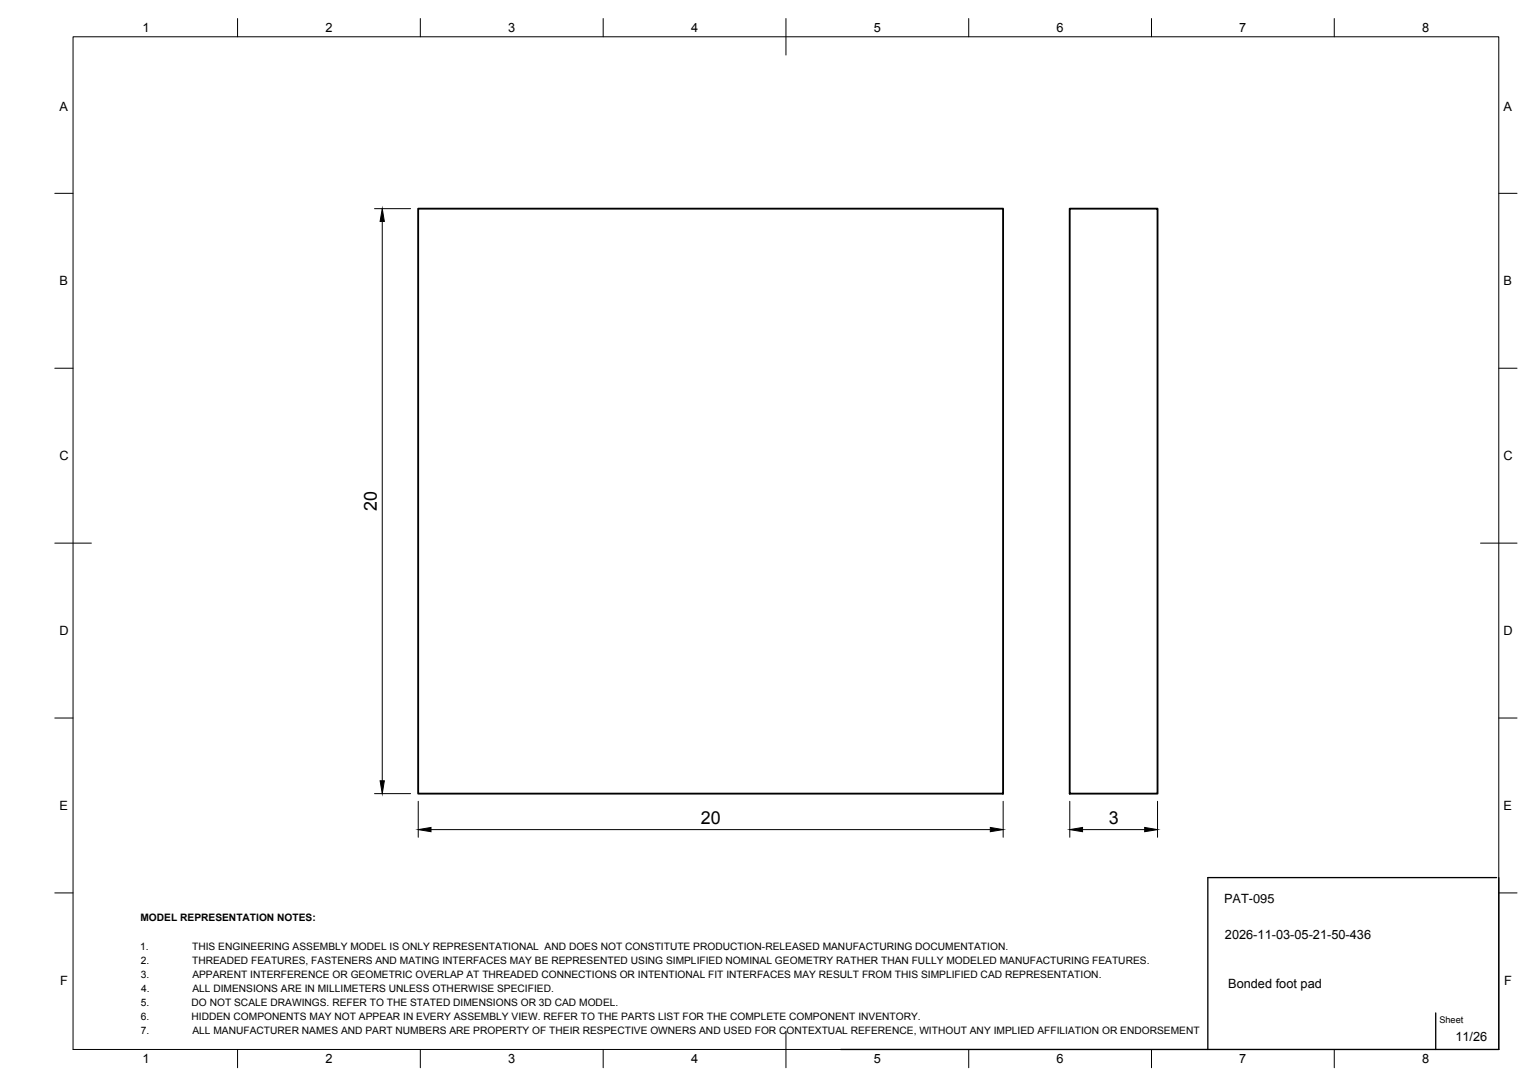
ISO-10303-21;
HEADER;
/* Generated by software containing ST-Developer
 * from STEP Tools, Inc. (www.steptools.com) 
 */

FILE_DESCRIPTION(
/* description */ ('Single-Axis Profile-Rail Linear Slide'),
/* implementation_level */ '2;1');

FILE_NAME(
/* name */ 'Bonded foot pad.step',
/* time_stamp */ '2026-10-27T10:47:43-07:00',
/* author */ (''),
/* organization */ (''),
/* preprocessor_version */ 'ST-DEVELOPER v20.2',
/* originating_system */ 'Autodesk Translation Framework v15.17.0.0',
/* authorisation */ '');

FILE_SCHEMA (('AUTOMOTIVE_DESIGN { 1 0 10303 214 3 1 1 }'));
ENDSEC;

DATA;
#10=MECHANICAL_DESIGN_GEOMETRIC_PRESENTATION_REPRESENTATION('',(#335),#14478);
#281=SHAPE_REPRESENTATION_RELATIONSHIP('SRR','None',#14611,#308);
#308=ADVANCED_BREP_SHAPE_REPRESENTATION('',(#362),#14455);
#335=STYLED_ITEM('',(#14824),#362);
#362=MANIFOLD_SOLID_BREP('Body1',#8595);
#624=PLANE('',#9156);
#625=PLANE('',#9157);
#626=PLANE('',#9158);
#627=PLANE('',#9159);
#628=PLANE('',#9160);
#629=PLANE('',#9161);
#1020=FACE_OUTER_BOUND('',#1519,.T.);
#1021=FACE_OUTER_BOUND('',#1520,.T.);
#1022=FACE_OUTER_BOUND('',#1521,.T.);
#1023=FACE_OUTER_BOUND('',#1522,.T.);
#1024=FACE_OUTER_BOUND('',#1523,.T.);
#1025=FACE_OUTER_BOUND('',#1524,.T.);
#1519=EDGE_LOOP('',(#6797,#6798,#6799,#6800));
#1520=EDGE_LOOP('',(#6801,#6802,#6803,#6804));
#1521=EDGE_LOOP('',(#6805,#6806,#6807,#6808));
#1522=EDGE_LOOP('',(#6809,#6810,#6811,#6812));
#1523=EDGE_LOOP('',(#6813,#6814,#6815,#6816));
#1524=EDGE_LOOP('',(#6817,#6818,#6819,#6820));
#2284=LINE('',#13008,#3255);
#2285=LINE('',#13010,#3256);
#2286=LINE('',#13012,#3257);
#2287=LINE('',#13013,#3258);
#2288=LINE('',#13016,#3259);
#2289=LINE('',#13018,#3260);
#2290=LINE('',#13019,#3261);
#2291=LINE('',#13022,#3262);
#2292=LINE('',#13024,#3263);
#2293=LINE('',#13025,#3264);
#2294=LINE('',#13027,#3265);
#2295=LINE('',#13028,#3266);
#3255=VECTOR('',#10541,1.);
#3256=VECTOR('',#10542,1.);
#3257=VECTOR('',#10543,1.);
#3258=VECTOR('',#10544,1.);
#3259=VECTOR('',#10547,1.);
#3260=VECTOR('',#10548,1.);
#3261=VECTOR('',#10549,1.);
#3262=VECTOR('',#10552,1.);
#3263=VECTOR('',#10553,1.);
#3264=VECTOR('',#10554,1.);
#3265=VECTOR('',#10557,1.);
#3266=VECTOR('',#10558,1.);
#4266=VERTEX_POINT('',#13006);
#4267=VERTEX_POINT('',#13007);
#4268=VERTEX_POINT('',#13009);
#4269=VERTEX_POINT('',#13011);
#4270=VERTEX_POINT('',#13015);
#4271=VERTEX_POINT('',#13017);
#4272=VERTEX_POINT('',#13021);
#4273=VERTEX_POINT('',#13023);
#5176=EDGE_CURVE('',#4266,#4267,#2284,.T.);
#5177=EDGE_CURVE('',#4267,#4268,#2285,.T.);
#5178=EDGE_CURVE('',#4269,#4268,#2286,.T.);
#5179=EDGE_CURVE('',#4266,#4269,#2287,.T.);
#5180=EDGE_CURVE('',#4270,#4266,#2288,.T.);
#5181=EDGE_CURVE('',#4271,#4269,#2289,.T.);
#5182=EDGE_CURVE('',#4270,#4271,#2290,.T.);
#5183=EDGE_CURVE('',#4272,#4270,#2291,.T.);
#5184=EDGE_CURVE('',#4273,#4271,#2292,.T.);
#5185=EDGE_CURVE('',#4272,#4273,#2293,.T.);
#5186=EDGE_CURVE('',#4267,#4272,#2294,.T.);
#5187=EDGE_CURVE('',#4268,#4273,#2295,.T.);
#6797=ORIENTED_EDGE('',*,*,#5176,.T.);
#6798=ORIENTED_EDGE('',*,*,#5177,.T.);
#6799=ORIENTED_EDGE('',*,*,#5178,.F.);
#6800=ORIENTED_EDGE('',*,*,#5179,.F.);
#6801=ORIENTED_EDGE('',*,*,#5180,.T.);
#6802=ORIENTED_EDGE('',*,*,#5179,.T.);
#6803=ORIENTED_EDGE('',*,*,#5181,.F.);
#6804=ORIENTED_EDGE('',*,*,#5182,.F.);
#6805=ORIENTED_EDGE('',*,*,#5183,.T.);
#6806=ORIENTED_EDGE('',*,*,#5182,.T.);
#6807=ORIENTED_EDGE('',*,*,#5184,.F.);
#6808=ORIENTED_EDGE('',*,*,#5185,.F.);
#6809=ORIENTED_EDGE('',*,*,#5186,.T.);
#6810=ORIENTED_EDGE('',*,*,#5185,.T.);
#6811=ORIENTED_EDGE('',*,*,#5187,.F.);
#6812=ORIENTED_EDGE('',*,*,#5177,.F.);
#6813=ORIENTED_EDGE('',*,*,#5187,.T.);
#6814=ORIENTED_EDGE('',*,*,#5184,.T.);
#6815=ORIENTED_EDGE('',*,*,#5181,.T.);
#6816=ORIENTED_EDGE('',*,*,#5178,.T.);
#6817=ORIENTED_EDGE('',*,*,#5186,.F.);
#6818=ORIENTED_EDGE('',*,*,#5176,.F.);
#6819=ORIENTED_EDGE('',*,*,#5180,.F.);
#6820=ORIENTED_EDGE('',*,*,#5183,.F.);
#8314=ADVANCED_FACE('',(#1020),#624,.T.);
#8315=ADVANCED_FACE('',(#1021),#625,.T.);
#8316=ADVANCED_FACE('',(#1022),#626,.T.);
#8317=ADVANCED_FACE('',(#1023),#627,.T.);
#8318=ADVANCED_FACE('',(#1024),#628,.T.);
#8319=ADVANCED_FACE('',(#1025),#629,.F.);
#8595=CLOSED_SHELL('',(#8314,#8315,#8316,#8317,#8318,#8319));
#9155=AXIS2_PLACEMENT_3D('',#13004,#10537,#10538);
#9156=AXIS2_PLACEMENT_3D('',#13005,#10539,#10540);
#9157=AXIS2_PLACEMENT_3D('',#13014,#10545,#10546);
#9158=AXIS2_PLACEMENT_3D('',#13020,#10550,#10551);
#9159=AXIS2_PLACEMENT_3D('',#13026,#10555,#10556);
#9160=AXIS2_PLACEMENT_3D('',#13029,#10559,#10560);
#9161=AXIS2_PLACEMENT_3D('',#13030,#10561,#10562);
#10537=DIRECTION('axis',(0.,0.,1.));
#10538=DIRECTION('refdir',(1.,0.,0.));
#10539=DIRECTION('center_axis',(0.,1.,0.));
#10540=DIRECTION('ref_axis',(-1.,0.,0.));
#10541=DIRECTION('',(-1.,0.,0.));
#10542=DIRECTION('',(0.,0.,1.));
#10543=DIRECTION('',(-1.,0.,0.));
#10544=DIRECTION('',(0.,0.,1.));
#10545=DIRECTION('center_axis',(1.,0.,0.));
#10546=DIRECTION('ref_axis',(0.,1.,0.));
#10547=DIRECTION('',(0.,1.,0.));
#10548=DIRECTION('',(0.,1.,0.));
#10549=DIRECTION('',(0.,0.,1.));
#10550=DIRECTION('center_axis',(0.,-1.,0.));
#10551=DIRECTION('ref_axis',(1.,0.,0.));
#10552=DIRECTION('',(1.,0.,0.));
#10553=DIRECTION('',(1.,0.,0.));
#10554=DIRECTION('',(0.,0.,1.));
#10555=DIRECTION('center_axis',(-1.,0.,0.));
#10556=DIRECTION('ref_axis',(0.,-1.,0.));
#10557=DIRECTION('',(0.,-1.,0.));
#10558=DIRECTION('',(0.,-1.,0.));
#10559=DIRECTION('center_axis',(0.,0.,1.));
#10560=DIRECTION('ref_axis',(1.,0.,0.));
#10561=DIRECTION('center_axis',(0.,0.,1.));
#10562=DIRECTION('ref_axis',(1.,0.,0.));
#13004=CARTESIAN_POINT('',(0.,0.,0.));
#13005=CARTESIAN_POINT('Origin',(4.,-2.5,-0.3));
#13006=CARTESIAN_POINT('',(4.,-2.5,-0.3));
#13007=CARTESIAN_POINT('',(2.,-2.5,-0.3));
#13008=CARTESIAN_POINT('',(4.,-2.5,-0.3));
#13009=CARTESIAN_POINT('',(2.,-2.5,0.));
#13010=CARTESIAN_POINT('',(2.,-2.5,-0.3));
#13011=CARTESIAN_POINT('',(4.,-2.5,0.));
#13012=CARTESIAN_POINT('',(4.,-2.5,0.));
#13013=CARTESIAN_POINT('',(4.,-2.5,-0.3));
#13014=CARTESIAN_POINT('Origin',(4.,-4.5,-0.3));
#13015=CARTESIAN_POINT('',(4.,-4.5,-0.3));
#13016=CARTESIAN_POINT('',(4.,-4.5,-0.3));
#13017=CARTESIAN_POINT('',(4.,-4.5,0.));
#13018=CARTESIAN_POINT('',(4.,-4.5,0.));
#13019=CARTESIAN_POINT('',(4.,-4.5,-0.3));
#13020=CARTESIAN_POINT('Origin',(2.,-4.5,-0.3));
#13021=CARTESIAN_POINT('',(2.,-4.5,-0.3));
#13022=CARTESIAN_POINT('',(2.,-4.5,-0.3));
#13023=CARTESIAN_POINT('',(2.,-4.5,0.));
#13024=CARTESIAN_POINT('',(2.,-4.5,0.));
#13025=CARTESIAN_POINT('',(2.,-4.5,-0.3));
#13026=CARTESIAN_POINT('Origin',(2.,-2.5,-0.3));
#13027=CARTESIAN_POINT('',(2.,-2.5,-0.3));
#13028=CARTESIAN_POINT('',(2.,-2.5,0.));
#13029=CARTESIAN_POINT('Origin',(3.,-3.5,0.));
#13030=CARTESIAN_POINT('Origin',(3.,-3.5,-0.3));
#14423=UNCERTAINTY_MEASURE_WITH_UNIT(LENGTH_MEASURE(0.001),#14479,
'DISTANCE_ACCURACY_VALUE',
'Maximum model space distance between geometric entities at asserted c
onnectivities');
#14446=UNCERTAINTY_MEASURE_WITH_UNIT(LENGTH_MEASURE(0.001),#14479,
'DISTANCE_ACCURACY_VALUE',
'Maximum model space distance between geometric entities at asserted c
onnectivities');
#14455=(
GEOMETRIC_REPRESENTATION_CONTEXT(3)
GLOBAL_UNCERTAINTY_ASSIGNED_CONTEXT((#14423))
GLOBAL_UNIT_ASSIGNED_CONTEXT((#14479,#14481,#14482))
REPRESENTATION_CONTEXT('','3D')
);
#14478=(
GEOMETRIC_REPRESENTATION_CONTEXT(3)
GLOBAL_UNCERTAINTY_ASSIGNED_CONTEXT((#14446))
GLOBAL_UNIT_ASSIGNED_CONTEXT((#14479,#14481,#14482))
REPRESENTATION_CONTEXT('','3D')
);
#14479=(
LENGTH_UNIT()
NAMED_UNIT(*)
SI_UNIT(.CENTI.,.METRE.)
);
#14481=(
NAMED_UNIT(*)
PLANE_ANGLE_UNIT()
SI_UNIT($,.RADIAN.)
);
#14482=(
NAMED_UNIT(*)
SI_UNIT($,.STERADIAN.)
SOLID_ANGLE_UNIT()
);
#14491=SHAPE_DEFINITION_REPRESENTATION(#14522,#14611);
#14522=PRODUCT_DEFINITION_SHAPE('',$,#14643);
#14611=SHAPE_REPRESENTATION('',(#9155),#14455);
#14634=PRODUCT_DEFINITION_CONTEXT('part definition',#14729,'design');
#14643=PRODUCT_DEFINITION('Bonded foot pad','Bonded foot pad',#14674,#14634);
#14674=PRODUCT_DEFINITION_FORMATION('',$,#14739);
#14729=APPLICATION_CONTEXT(
'Core Data for Automotive Mechanical Design Process');
#14730=PRODUCT_CONTEXT('part definition',#14729,'mechanical');
#14739=PRODUCT('Bonded foot pad','Bonded foot pad','Bonded foot pad',(#14730));
#14818=COLOUR_RGB('Sky Blue',0.24,0.69,0.87);
#14819=FILL_AREA_STYLE_COLOUR('',#14818);
#14820=FILL_AREA_STYLE('',(#14819));
#14821=SURFACE_STYLE_FILL_AREA(#14820);
#14822=SURFACE_SIDE_STYLE('',(#14821));
#14823=SURFACE_STYLE_USAGE(.BOTH.,#14822);
#14824=PRESENTATION_STYLE_ASSIGNMENT((#14823));
ENDSEC;
END-ISO-10303-21;
